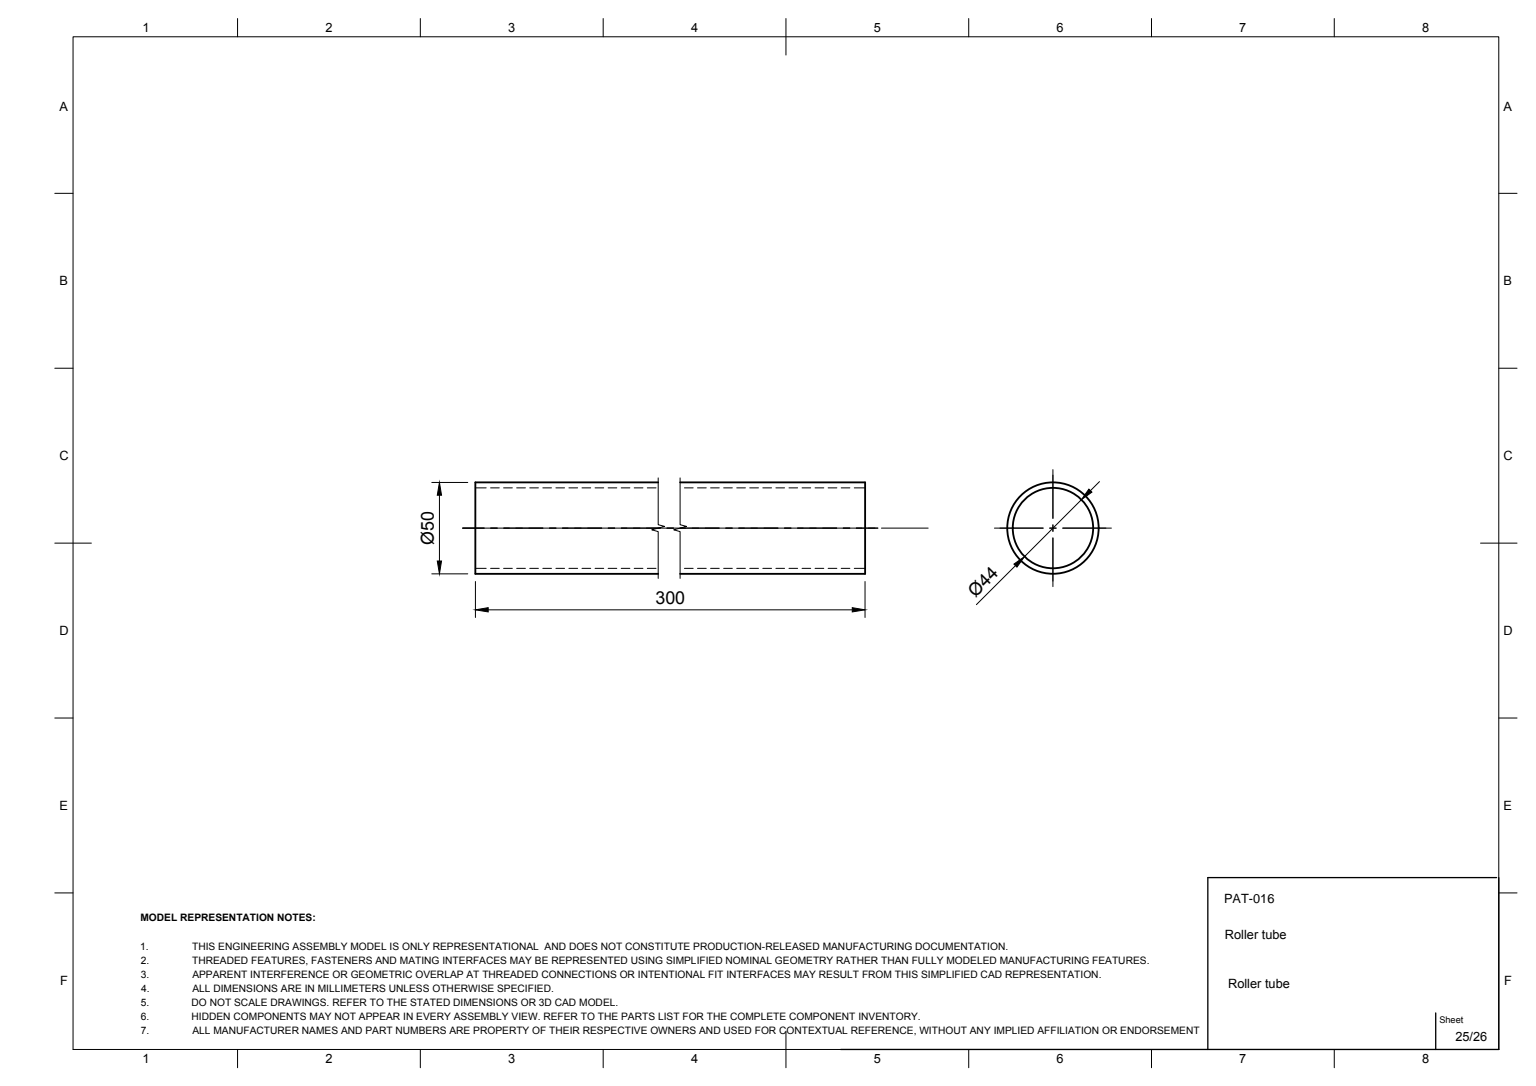
ISO-10303-21;
HEADER;
/* Generated by software containing ST-Developer
 * from STEP Tools, Inc. (www.steptools.com) 
 */

FILE_DESCRIPTION(
/* description */ ('Bracket-mounted idler roller'),
/* implementation_level */ '2;1');

FILE_NAME(
/* name */ 'Roller tube.step',
/* time_stamp */ '2026-10-28T03:26:42-07:00',
/* author */ (''),
/* organization */ (''),
/* preprocessor_version */ 'ST-DEVELOPER v20.2',
/* originating_system */ 'Autodesk Translation Framework v15.17.0.0',
/* authorisation */ '');

FILE_SCHEMA (('AUTOMOTIVE_DESIGN { 1 0 10303 214 3 1 1 }'));
ENDSEC;

DATA;
#10=MECHANICAL_DESIGN_GEOMETRIC_PRESENTATION_REPRESENTATION('',(#306),#6241);
#256=SHAPE_REPRESENTATION_RELATIONSHIP('SRR','None',#6362,#277);
#277=ADVANCED_BREP_SHAPE_REPRESENTATION('',(#334),#6238);
#306=STYLED_ITEM('',(#6524),#334);
#334=MANIFOLD_SOLID_BREP('Body1',#3209);
#404=FACE_BOUND('',#940,.T.);
#405=FACE_BOUND('',#942,.T.);
#501=PLANE('',#3798);
#502=PLANE('',#3799);
#678=FACE_OUTER_BOUND('',#937,.T.);
#679=FACE_OUTER_BOUND('',#938,.T.);
#680=FACE_OUTER_BOUND('',#939,.T.);
#681=FACE_OUTER_BOUND('',#941,.T.);
#937=EDGE_LOOP('',(#2816,#2817,#2818,#2819));
#938=EDGE_LOOP('',(#2820,#2821,#2822,#2823));
#939=EDGE_LOOP('',(#2824));
#940=EDGE_LOOP('',(#2825));
#941=EDGE_LOOP('',(#2826));
#942=EDGE_LOOP('',(#2827));
#1129=LINE('',#6032,#1311);
#1130=LINE('',#6038,#1312);
#1311=VECTOR('',#4734,2.2);
#1312=VECTOR('',#4741,2.5);
#1500=CIRCLE('',#3793,2.2);
#1501=CIRCLE('',#3794,2.2);
#1502=CIRCLE('',#3796,2.5);
#1503=CIRCLE('',#3797,2.5);
#1749=VERTEX_POINT('',#6029);
#1750=VERTEX_POINT('',#6031);
#1751=VERTEX_POINT('',#6035);
#1752=VERTEX_POINT('',#6037);
#2110=EDGE_CURVE('',#1749,#1749,#1500,.T.);
#2111=EDGE_CURVE('',#1749,#1750,#1129,.T.);
#2112=EDGE_CURVE('',#1750,#1750,#1501,.T.);
#2113=EDGE_CURVE('',#1751,#1751,#1502,.T.);
#2114=EDGE_CURVE('',#1751,#1752,#1130,.T.);
#2115=EDGE_CURVE('',#1752,#1752,#1503,.T.);
#2816=ORIENTED_EDGE('',*,*,#2110,.F.);
#2817=ORIENTED_EDGE('',*,*,#2111,.T.);
#2818=ORIENTED_EDGE('',*,*,#2112,.T.);
#2819=ORIENTED_EDGE('',*,*,#2111,.F.);
#2820=ORIENTED_EDGE('',*,*,#2113,.F.);
#2821=ORIENTED_EDGE('',*,*,#2114,.T.);
#2822=ORIENTED_EDGE('',*,*,#2115,.T.);
#2823=ORIENTED_EDGE('',*,*,#2114,.F.);
#2824=ORIENTED_EDGE('',*,*,#2113,.T.);
#2825=ORIENTED_EDGE('',*,*,#2110,.T.);
#2826=ORIENTED_EDGE('',*,*,#2115,.F.);
#2827=ORIENTED_EDGE('',*,*,#2112,.F.);
#2981=CYLINDRICAL_SURFACE('',#3792,2.2);
#2982=CYLINDRICAL_SURFACE('',#3795,2.5);
#3153=ADVANCED_FACE('',(#678),#2981,.F.);
#3154=ADVANCED_FACE('',(#679),#2982,.T.);
#3155=ADVANCED_FACE('',(#680,#404),#501,.T.);
#3156=ADVANCED_FACE('',(#681,#405),#502,.F.);
#3209=CLOSED_SHELL('',(#3153,#3154,#3155,#3156));
#3791=AXIS2_PLACEMENT_3D('',#6027,#4728,#4729);
#3792=AXIS2_PLACEMENT_3D('',#6028,#4730,#4731);
#3793=AXIS2_PLACEMENT_3D('',#6030,#4732,#4733);
#3794=AXIS2_PLACEMENT_3D('',#6033,#4735,#4736);
#3795=AXIS2_PLACEMENT_3D('',#6034,#4737,#4738);
#3796=AXIS2_PLACEMENT_3D('',#6036,#4739,#4740);
#3797=AXIS2_PLACEMENT_3D('',#6039,#4742,#4743);
#3798=AXIS2_PLACEMENT_3D('',#6040,#4744,#4745);
#3799=AXIS2_PLACEMENT_3D('',#6041,#4746,#4747);
#4728=DIRECTION('axis',(0.,0.,1.));
#4729=DIRECTION('refdir',(1.,0.,0.));
#4730=DIRECTION('center_axis',(0.,1.,0.));
#4731=DIRECTION('ref_axis',(1.,0.,0.));
#4732=DIRECTION('center_axis',(0.,-1.,0.));
#4733=DIRECTION('ref_axis',(1.,0.,0.));
#4734=DIRECTION('',(0.,-1.,0.));
#4735=DIRECTION('center_axis',(0.,-1.,0.));
#4736=DIRECTION('ref_axis',(1.,0.,0.));
#4737=DIRECTION('center_axis',(0.,1.,0.));
#4738=DIRECTION('ref_axis',(1.,0.,0.));
#4739=DIRECTION('center_axis',(0.,1.,0.));
#4740=DIRECTION('ref_axis',(1.,0.,0.));
#4741=DIRECTION('',(0.,-1.,0.));
#4742=DIRECTION('center_axis',(0.,1.,0.));
#4743=DIRECTION('ref_axis',(1.,0.,0.));
#4744=DIRECTION('center_axis',(0.,1.,0.));
#4745=DIRECTION('ref_axis',(1.,0.,0.));
#4746=DIRECTION('center_axis',(0.,1.,0.));
#4747=DIRECTION('ref_axis',(1.,0.,0.));
#6027=CARTESIAN_POINT('',(0.,0.,0.));
#6028=CARTESIAN_POINT('Origin',(0.,0.,4.5));
#6029=CARTESIAN_POINT('',(-2.2,30.,4.5));
#6030=CARTESIAN_POINT('Origin',(0.,30.,4.5));
#6031=CARTESIAN_POINT('',(-2.2,0.,4.5));
#6032=CARTESIAN_POINT('',(-2.2,0.,4.5));
#6033=CARTESIAN_POINT('Origin',(0.,0.,4.5));
#6034=CARTESIAN_POINT('Origin',(0.,0.,4.5));
#6035=CARTESIAN_POINT('',(-2.5,30.,4.5));
#6036=CARTESIAN_POINT('Origin',(0.,30.,4.5));
#6037=CARTESIAN_POINT('',(-2.5,0.,4.5));
#6038=CARTESIAN_POINT('',(-2.5,0.,4.5));
#6039=CARTESIAN_POINT('Origin',(0.,0.,4.5));
#6040=CARTESIAN_POINT('Origin',(0.,30.,4.5));
#6041=CARTESIAN_POINT('Origin',(0.,0.,4.5));
#6212=UNCERTAINTY_MEASURE_WITH_UNIT(LENGTH_MEASURE(0.001),#6242,
'DISTANCE_ACCURACY_VALUE',
'Maximum model space distance between geometric entities at asserted c
onnectivities');
#6215=UNCERTAINTY_MEASURE_WITH_UNIT(LENGTH_MEASURE(0.001),#6242,
'DISTANCE_ACCURACY_VALUE',
'Maximum model space distance between geometric entities at asserted c
onnectivities');
#6238=(
GEOMETRIC_REPRESENTATION_CONTEXT(3)
GLOBAL_UNCERTAINTY_ASSIGNED_CONTEXT((#6212))
GLOBAL_UNIT_ASSIGNED_CONTEXT((#6242,#6244,#6245))
REPRESENTATION_CONTEXT('','3D')
);
#6241=(
GEOMETRIC_REPRESENTATION_CONTEXT(3)
GLOBAL_UNCERTAINTY_ASSIGNED_CONTEXT((#6215))
GLOBAL_UNIT_ASSIGNED_CONTEXT((#6242,#6244,#6245))
REPRESENTATION_CONTEXT('','3D')
);
#6242=(
LENGTH_UNIT()
NAMED_UNIT(*)
SI_UNIT(.CENTI.,.METRE.)
);
#6244=(
NAMED_UNIT(*)
PLANE_ANGLE_UNIT()
SI_UNIT($,.RADIAN.)
);
#6245=(
NAMED_UNIT(*)
SI_UNIT($,.STERADIAN.)
SOLID_ANGLE_UNIT()
);
#6268=SHAPE_DEFINITION_REPRESENTATION(#6298,#6362);
#6298=PRODUCT_DEFINITION_SHAPE('',$,#6388);
#6362=SHAPE_REPRESENTATION('',(#3791),#6238);
#6365=PRODUCT_DEFINITION_CONTEXT('part definition',#6442,'design');
#6388=PRODUCT_DEFINITION('Roller tube','Roller tube',#6413,#6365);
#6413=PRODUCT_DEFINITION_FORMATION('',$,#6466);
#6442=APPLICATION_CONTEXT(
'Core Data for Automotive Mechanical Design Process');
#6443=PRODUCT_CONTEXT('part definition',#6442,'mechanical');
#6466=PRODUCT('Roller tube','Roller tube','Roller tube',(#6443));
#6518=COLOUR_RGB('Light Blue',0.38,0.62,0.78);
#6519=FILL_AREA_STYLE_COLOUR('',#6518);
#6520=FILL_AREA_STYLE('',(#6519));
#6521=SURFACE_STYLE_FILL_AREA(#6520);
#6522=SURFACE_SIDE_STYLE('',(#6521));
#6523=SURFACE_STYLE_USAGE(.BOTH.,#6522);
#6524=PRESENTATION_STYLE_ASSIGNMENT((#6523));
ENDSEC;
END-ISO-10303-21;
